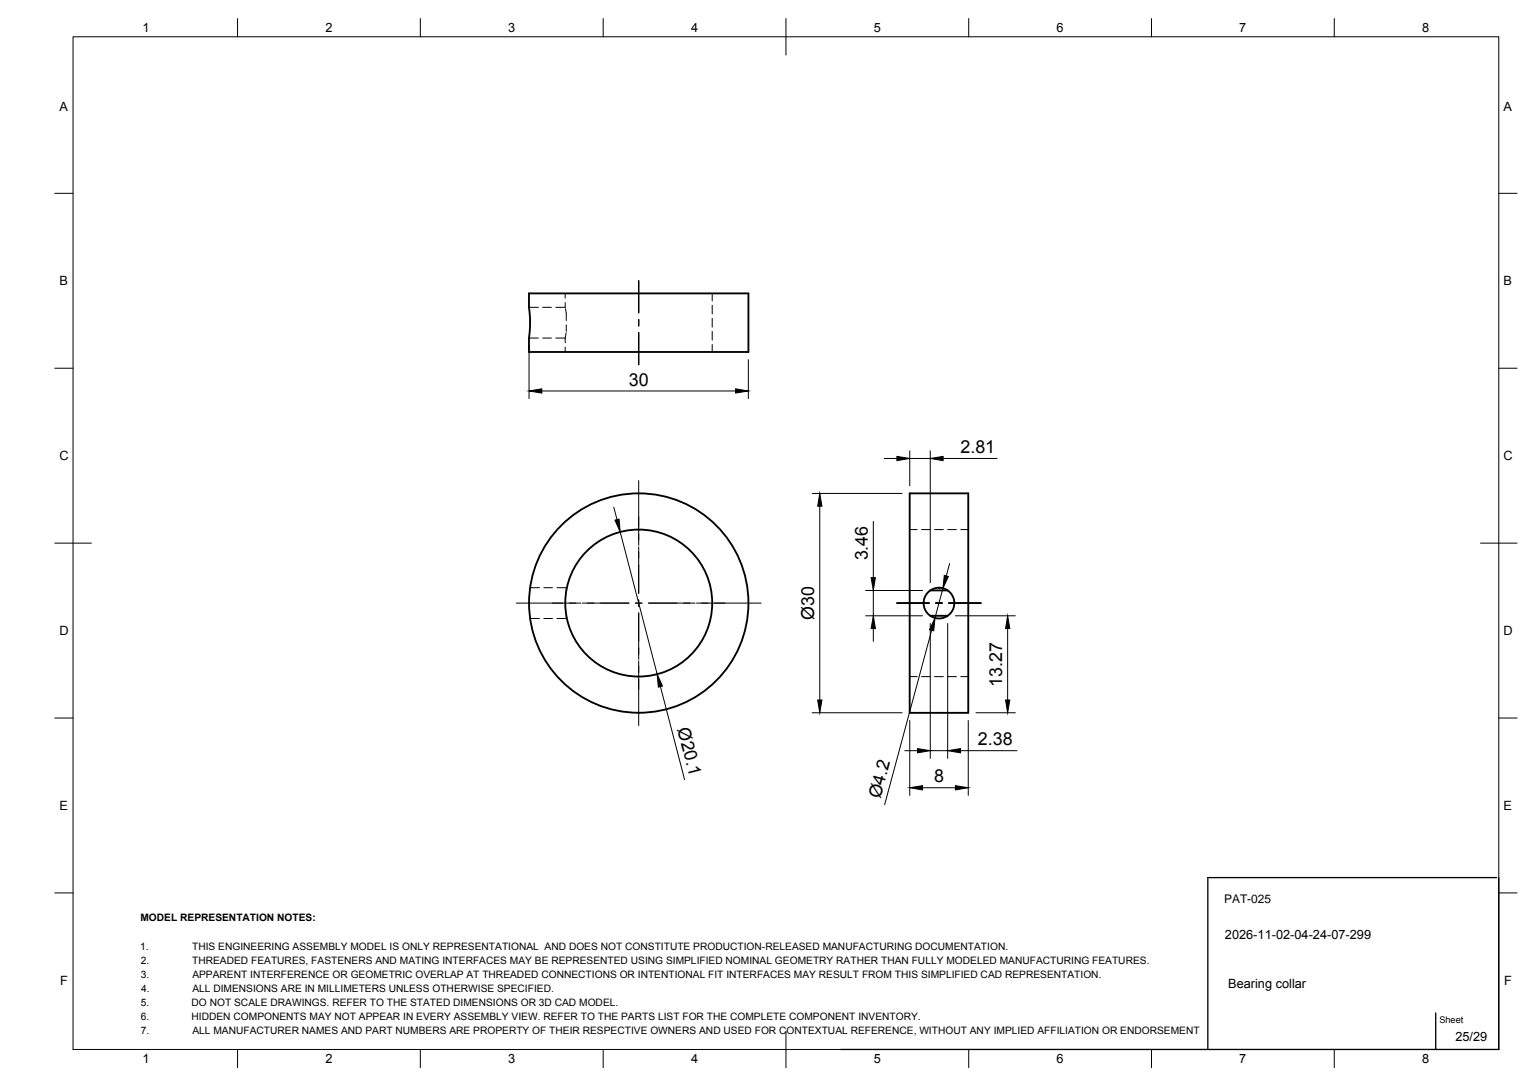
ISO-10303-21;
HEADER;
/* Generated by software containing ST-Developer
 * from STEP Tools, Inc. (www.steptools.com) 
 */

FILE_DESCRIPTION(
/* description */ ('Counter shaft with two pulleys and keyed hub'),
/* implementation_level */ '2;1');

FILE_NAME(
/* name */ 'Bearing collar.step',
/* time_stamp */ '2026-10-27T10:46:10-07:00',
/* author */ (''),
/* organization */ (''),
/* preprocessor_version */ 'ST-DEVELOPER v20.2',
/* originating_system */ 'Autodesk Translation Framework v15.17.0.0',
/* authorisation */ '');

FILE_SCHEMA (('AUTOMOTIVE_DESIGN { 1 0 10303 214 3 1 1 }'));
ENDSEC;

DATA;
#10=MECHANICAL_DESIGN_GEOMETRIC_PRESENTATION_REPRESENTATION('',(#309),#10821);
#212=B_SPLINE_CURVE_WITH_KNOTS('',3,(#9516,#9517,#9518,#9519,#9520,#9521,
#9522,#9523,#9524,#9525,#9526,#9527,#9528,#9529),.UNSPECIFIED.,.F.,.F.,
(4,2,2,2,2,2,4),(0.75600573798702,0.793568827564647,0.872922520054201,0.952276212543756,
1.03162990503331,1.11098359752287,1.14854668710049),.UNSPECIFIED.);
#213=B_SPLINE_CURVE_WITH_KNOTS('',3,(#9535,#9536,#9537,#9538,#9539,#9540,
#9541,#9542,#9543,#9544,#9545,#9546,#9547,#9548,#9549,#9550,#9551,#9552),
 .UNSPECIFIED.,.F.,.F.,(4,2,2,2,2,2,2,2,4),(0.,0.079216580773363,0.158433161546726,
0.23764869707457,0.316864232602414,0.396079768130259,0.475295303658103,
0.554511884431466,0.633728465204829),.UNSPECIFIED.);
#214=B_SPLINE_CURVE_WITH_KNOTS('',3,(#9553,#9554,#9555,#9556,#9557,#9558,
#9559,#9560,#9561,#9562,#9563,#9564,#9565,#9566,#9567,#9568,#9569,#9570),
 .UNSPECIFIED.,.F.,.F.,(4,2,2,2,2,2,2,2,4),(0.633728465204829,0.712945045978192,
0.792161626751555,0.871377162279399,0.950592697807244,1.02980823333509,
1.10902376886293,1.18824034963629,1.26745693040966),.UNSPECIFIED.);
#215=B_SPLINE_CURVE_WITH_KNOTS('',3,(#9573,#9574,#9575,#9576,#9577,#9578,
#9579,#9580,#9581,#9582,#9583,#9584,#9585,#9586),.UNSPECIFIED.,.F.,.F.,
(4,2,2,2,2,2,4),(0.121154929624515,0.158718019202143,0.238071711691697,
0.317425404181252,0.396779096670807,0.476132789160362,0.513695878737989),
 .UNSPECIFIED.);
#258=SHAPE_REPRESENTATION_RELATIONSHIP('SRR','None',#10946,#283);
#283=ADVANCED_BREP_SHAPE_REPRESENTATION('',(#334),#10814);
#309=STYLED_ITEM('',(#11135),#334);
#334=MANIFOLD_SOLID_BREP('Body1',#5593);
#409=FACE_BOUND('',#1130,.T.);
#410=FACE_BOUND('',#1132,.T.);
#411=FACE_BOUND('',#1134,.T.);
#412=FACE_BOUND('',#1136,.T.);
#532=PLANE('',#6178);
#533=PLANE('',#6183);
#534=PLANE('',#6190);
#535=PLANE('',#6191);
#743=FACE_OUTER_BOUND('',#1126,.T.);
#744=FACE_OUTER_BOUND('',#1127,.T.);
#745=FACE_OUTER_BOUND('',#1128,.T.);
#746=FACE_OUTER_BOUND('',#1129,.T.);
#747=FACE_OUTER_BOUND('',#1131,.T.);
#748=FACE_OUTER_BOUND('',#1133,.T.);
#749=FACE_OUTER_BOUND('',#1135,.T.);
#1126=EDGE_LOOP('',(#4269,#4270));
#1127=EDGE_LOOP('',(#4271,#4272,#4273,#4274,#4275,#4276,#4277,#4278,#4279));
#1128=EDGE_LOOP('',(#4280,#4281,#4282));
#1129=EDGE_LOOP('',(#4283,#4284,#4285,#4286));
#1130=EDGE_LOOP('',(#4287,#4288,#4289,#4290));
#1131=EDGE_LOOP('',(#4291,#4292,#4293,#4294));
#1132=EDGE_LOOP('',(#4295,#4296));
#1133=EDGE_LOOP('',(#4297));
#1134=EDGE_LOOP('',(#4298));
#1135=EDGE_LOOP('',(#4299));
#1136=EDGE_LOOP('',(#4300));
#1495=LINE('',#9512,#1884);
#1496=LINE('',#9533,#1885);
#1497=LINE('',#9588,#1886);
#1498=LINE('',#9593,#1887);
#1499=LINE('',#9599,#1888);
#1884=VECTOR('',#7351,1.);
#1885=VECTOR('',#7358,0.21);
#1886=VECTOR('',#7363,1.);
#1887=VECTOR('',#7368,1.005);
#1888=VECTOR('',#7375,1.5);
#2189=CIRCLE('',#6179,0.21);
#2190=CIRCLE('',#6181,0.21);
#2191=CIRCLE('',#6182,0.21);
#2192=CIRCLE('',#6185,1.005);
#2193=CIRCLE('',#6186,1.005);
#2194=CIRCLE('',#6188,1.5);
#2195=CIRCLE('',#6189,1.5);
#2604=VERTEX_POINT('',#9510);
#2605=VERTEX_POINT('',#9511);
#2606=VERTEX_POINT('',#9515);
#2607=VERTEX_POINT('',#9530);
#2608=VERTEX_POINT('',#9532);
#2609=VERTEX_POINT('',#9534);
#2610=VERTEX_POINT('',#9571);
#2611=VERTEX_POINT('',#9590);
#2612=VERTEX_POINT('',#9592);
#2613=VERTEX_POINT('',#9596);
#2614=VERTEX_POINT('',#9598);
#3207=EDGE_CURVE('',#2604,#2605,#1495,.T.);
#3208=EDGE_CURVE('',#2604,#2605,#2189,.T.);
#3209=EDGE_CURVE('',#2606,#2604,#212,.T.);
#3210=EDGE_CURVE('',#2607,#2606,#2190,.T.);
#3211=EDGE_CURVE('',#2607,#2608,#1496,.T.);
#3212=EDGE_CURVE('',#2609,#2608,#213,.T.);
#3213=EDGE_CURVE('',#2608,#2609,#214,.T.);
#3214=EDGE_CURVE('',#2610,#2607,#2191,.T.);
#3215=EDGE_CURVE('',#2605,#2610,#215,.T.);
#3216=EDGE_CURVE('',#2610,#2606,#1497,.T.);
#3217=EDGE_CURVE('',#2611,#2611,#2192,.T.);
#3218=EDGE_CURVE('',#2611,#2612,#1498,.T.);
#3219=EDGE_CURVE('',#2612,#2612,#2193,.T.);
#3220=EDGE_CURVE('',#2613,#2613,#2194,.T.);
#3221=EDGE_CURVE('',#2613,#2614,#1499,.T.);
#3222=EDGE_CURVE('',#2614,#2614,#2195,.T.);
#4269=ORIENTED_EDGE('',*,*,#3207,.F.);
#4270=ORIENTED_EDGE('',*,*,#3208,.T.);
#4271=ORIENTED_EDGE('',*,*,#3209,.F.);
#4272=ORIENTED_EDGE('',*,*,#3210,.F.);
#4273=ORIENTED_EDGE('',*,*,#3211,.T.);
#4274=ORIENTED_EDGE('',*,*,#3212,.F.);
#4275=ORIENTED_EDGE('',*,*,#3213,.F.);
#4276=ORIENTED_EDGE('',*,*,#3211,.F.);
#4277=ORIENTED_EDGE('',*,*,#3214,.F.);
#4278=ORIENTED_EDGE('',*,*,#3215,.F.);
#4279=ORIENTED_EDGE('',*,*,#3208,.F.);
#4280=ORIENTED_EDGE('',*,*,#3216,.F.);
#4281=ORIENTED_EDGE('',*,*,#3214,.T.);
#4282=ORIENTED_EDGE('',*,*,#3210,.T.);
#4283=ORIENTED_EDGE('',*,*,#3217,.F.);
#4284=ORIENTED_EDGE('',*,*,#3218,.T.);
#4285=ORIENTED_EDGE('',*,*,#3219,.T.);
#4286=ORIENTED_EDGE('',*,*,#3218,.F.);
#4287=ORIENTED_EDGE('',*,*,#3215,.T.);
#4288=ORIENTED_EDGE('',*,*,#3216,.T.);
#4289=ORIENTED_EDGE('',*,*,#3209,.T.);
#4290=ORIENTED_EDGE('',*,*,#3207,.T.);
#4291=ORIENTED_EDGE('',*,*,#3220,.F.);
#4292=ORIENTED_EDGE('',*,*,#3221,.T.);
#4293=ORIENTED_EDGE('',*,*,#3222,.T.);
#4294=ORIENTED_EDGE('',*,*,#3221,.F.);
#4295=ORIENTED_EDGE('',*,*,#3212,.T.);
#4296=ORIENTED_EDGE('',*,*,#3213,.T.);
#4297=ORIENTED_EDGE('',*,*,#3220,.T.);
#4298=ORIENTED_EDGE('',*,*,#3217,.T.);
#4299=ORIENTED_EDGE('',*,*,#3222,.F.);
#4300=ORIENTED_EDGE('',*,*,#3219,.F.);
#5162=CYLINDRICAL_SURFACE('',#6180,0.21);
#5163=CYLINDRICAL_SURFACE('',#6184,1.005);
#5164=CYLINDRICAL_SURFACE('',#6187,1.5);
#5414=ADVANCED_FACE('',(#743),#532,.T.);
#5415=ADVANCED_FACE('',(#744),#5162,.F.);
#5416=ADVANCED_FACE('',(#745),#533,.T.);
#5417=ADVANCED_FACE('',(#746,#409),#5163,.F.);
#5418=ADVANCED_FACE('',(#747,#410),#5164,.T.);
#5419=ADVANCED_FACE('',(#748,#411),#534,.T.);
#5420=ADVANCED_FACE('',(#749,#412),#535,.F.);
#5593=CLOSED_SHELL('',(#5414,#5415,#5416,#5417,#5418,#5419,#5420));
#6177=AXIS2_PLACEMENT_3D('',#9508,#7347,#7348);
#6178=AXIS2_PLACEMENT_3D('',#9509,#7349,#7350);
#6179=AXIS2_PLACEMENT_3D('',#9513,#7352,#7353);
#6180=AXIS2_PLACEMENT_3D('',#9514,#7354,#7355);
#6181=AXIS2_PLACEMENT_3D('',#9531,#7356,#7357);
#6182=AXIS2_PLACEMENT_3D('',#9572,#7359,#7360);
#6183=AXIS2_PLACEMENT_3D('',#9587,#7361,#7362);
#6184=AXIS2_PLACEMENT_3D('',#9589,#7364,#7365);
#6185=AXIS2_PLACEMENT_3D('',#9591,#7366,#7367);
#6186=AXIS2_PLACEMENT_3D('',#9594,#7369,#7370);
#6187=AXIS2_PLACEMENT_3D('',#9595,#7371,#7372);
#6188=AXIS2_PLACEMENT_3D('',#9597,#7373,#7374);
#6189=AXIS2_PLACEMENT_3D('',#9600,#7376,#7377);
#6190=AXIS2_PLACEMENT_3D('',#9601,#7378,#7379);
#6191=AXIS2_PLACEMENT_3D('',#9602,#7380,#7381);
#7347=DIRECTION('axis',(0.,0.,1.));
#7348=DIRECTION('refdir',(1.,0.,0.));
#7349=DIRECTION('center_axis',(0.,0.,1.));
#7350=DIRECTION('ref_axis',(1.,0.,0.));
#7351=DIRECTION('',(0.,1.,0.));
#7352=DIRECTION('center_axis',(0.,0.,1.));
#7353=DIRECTION('ref_axis',(1.,0.,0.));
#7354=DIRECTION('center_axis',(0.,0.,1.));
#7355=DIRECTION('ref_axis',(1.,0.,0.));
#7356=DIRECTION('center_axis',(0.,0.,1.));
#7357=DIRECTION('ref_axis',(1.,0.,0.));
#7358=DIRECTION('',(0.,0.,1.));
#7359=DIRECTION('center_axis',(0.,0.,1.));
#7360=DIRECTION('ref_axis',(1.,0.,0.));
#7361=DIRECTION('center_axis',(0.,0.,1.));
#7362=DIRECTION('ref_axis',(1.,0.,0.));
#7363=DIRECTION('',(0.,-1.,0.));
#7364=DIRECTION('center_axis',(0.,1.,0.));
#7365=DIRECTION('ref_axis',(1.,0.,0.));
#7366=DIRECTION('center_axis',(0.,-1.,0.));
#7367=DIRECTION('ref_axis',(1.,0.,0.));
#7368=DIRECTION('',(0.,-1.,0.));
#7369=DIRECTION('center_axis',(0.,-1.,0.));
#7370=DIRECTION('ref_axis',(1.,0.,0.));
#7371=DIRECTION('center_axis',(0.,1.,0.));
#7372=DIRECTION('ref_axis',(1.,0.,0.));
#7373=DIRECTION('center_axis',(0.,1.,0.));
#7374=DIRECTION('ref_axis',(1.,0.,0.));
#7375=DIRECTION('',(0.,-1.,0.));
#7376=DIRECTION('center_axis',(0.,1.,0.));
#7377=DIRECTION('ref_axis',(1.,0.,0.));
#7378=DIRECTION('center_axis',(0.,1.,0.));
#7379=DIRECTION('ref_axis',(1.,0.,0.));
#7380=DIRECTION('center_axis',(0.,1.,0.));
#7381=DIRECTION('ref_axis',(1.,0.,0.));
#9508=CARTESIAN_POINT('',(0.,0.,0.));
#9509=CARTESIAN_POINT('Origin',(0.,-1.25,5.52));
#9510=CARTESIAN_POINT('',(0.172988438920056,-1.36905880899792,5.52));
#9511=CARTESIAN_POINT('',(0.172988438920056,-1.13094119100209,5.52));
#9512=CARTESIAN_POINT('',(0.172988438920056,-1.65,5.52));
#9513=CARTESIAN_POINT('Origin',(0.,-1.25,5.52));
#9514=CARTESIAN_POINT('Origin',(0.,-1.25,5.52));
#9515=CARTESIAN_POINT('',(-0.172988438920056,-1.36905880899792,5.52));
#9516=CARTESIAN_POINT('Ctrl Pts',(-0.172988438920056,-1.36905880899792,
5.52));
#9517=CARTESIAN_POINT('Ctrl Pts',(-0.165594865311314,-1.37980142239529,
5.52129192197638));
#9518=CARTESIAN_POINT('Ctrl Pts',(-0.157297138725606,-1.38968770937274,
5.52265394943905));
#9519=CARTESIAN_POINT('Ctrl Pts',(-0.129892073845076,-1.41709277425327,
5.5267480843909));
#9520=CARTESIAN_POINT('Ctrl Pts',(-0.106330167759284,-1.43324205633295,
5.52969589327638));
#9521=CARTESIAN_POINT('Ctrl Pts',(-0.0546129046324105,-1.45469779396491,
5.53385029472357));
#9522=CARTESIAN_POINT('Ctrl Pts',(-0.0264512308298517,-1.46,5.535));
#9523=CARTESIAN_POINT('Ctrl Pts',(0.0264512308298516,-1.46,5.535));
#9524=CARTESIAN_POINT('Ctrl Pts',(0.0546129046324104,-1.45469779396491,
5.53385029472357));
#9525=CARTESIAN_POINT('Ctrl Pts',(0.106330167759284,-1.43324205633295,5.52969589327638));
#9526=CARTESIAN_POINT('Ctrl Pts',(0.129892073845076,-1.41709277425327,5.5267480843909));
#9527=CARTESIAN_POINT('Ctrl Pts',(0.157297138725606,-1.38968770937274,5.52265394943905));
#9528=CARTESIAN_POINT('Ctrl Pts',(0.165594865311314,-1.37980142239529,5.52129192197638));
#9529=CARTESIAN_POINT('Ctrl Pts',(0.172988438920056,-1.36905880899792,5.52));
#9530=CARTESIAN_POINT('',(-0.21,-1.25,5.52));
#9531=CARTESIAN_POINT('Origin',(0.,-1.25,5.52));
#9532=CARTESIAN_POINT('',(-0.21,-1.25,6.01522725533839));
#9533=CARTESIAN_POINT('',(-0.21,-1.25,5.52));
#9534=CARTESIAN_POINT('',(0.21,-1.25,6.01522725533839));
#9535=CARTESIAN_POINT('Ctrl Pts',(0.21,-1.25,6.01522725533839));
#9536=CARTESIAN_POINT('Ctrl Pts',(0.21,-1.27640552692445,6.01522725533839));
#9537=CARTESIAN_POINT('Ctrl Pts',(0.204715737269596,-1.30454707409071,6.01600415954412));
#9538=CARTESIAN_POINT('Ctrl Pts',(0.183273763036331,-1.35627626890513,6.01880073282317));
#9539=CARTESIAN_POINT('Ctrl Pts',(0.167117923970394,-1.37986692412796,6.02077897157582));
#9540=CARTESIAN_POINT('Ctrl Pts',(0.129867169887369,-1.41711767821098,6.02448481141327));
#9541=CARTESIAN_POINT('Ctrl Pts',(0.106276408305765,-1.43327371000135,6.02645455657129));
#9542=CARTESIAN_POINT('Ctrl Pts',(0.0545468514059002,-1.45471582482622,
6.02923165515645));
#9543=CARTESIAN_POINT('Ctrl Pts',(0.0264051785092814,-1.46,6.03));
#9544=CARTESIAN_POINT('Ctrl Pts',(-0.0264051785092814,-1.46,6.03));
#9545=CARTESIAN_POINT('Ctrl Pts',(-0.0545468514059001,-1.45471582482622,
6.02923165515645));
#9546=CARTESIAN_POINT('Ctrl Pts',(-0.106276408305765,-1.43327371000135,
6.02645455657129));
#9547=CARTESIAN_POINT('Ctrl Pts',(-0.129867169887369,-1.41711767821098,
6.02448481141327));
#9548=CARTESIAN_POINT('Ctrl Pts',(-0.167117923970394,-1.37986692412796,
6.02077897157582));
#9549=CARTESIAN_POINT('Ctrl Pts',(-0.183273763036331,-1.35627626890513,
6.01880073282317));
#9550=CARTESIAN_POINT('Ctrl Pts',(-0.204715737269596,-1.30454707409071,
6.01600415954412));
#9551=CARTESIAN_POINT('Ctrl Pts',(-0.21,-1.27640552692445,6.01522725533839));
#9552=CARTESIAN_POINT('Ctrl Pts',(-0.21,-1.25,6.01522725533839));
#9553=CARTESIAN_POINT('Ctrl Pts',(-0.21,-1.25,6.01522725533839));
#9554=CARTESIAN_POINT('Ctrl Pts',(-0.21,-1.22359447307555,6.01522725533839));
#9555=CARTESIAN_POINT('Ctrl Pts',(-0.204715737269596,-1.19545292590929,
6.01600415954412));
#9556=CARTESIAN_POINT('Ctrl Pts',(-0.183273763036331,-1.14372373109487,
6.01880073282317));
#9557=CARTESIAN_POINT('Ctrl Pts',(-0.167117923970394,-1.12013307587204,
6.02077897157582));
#9558=CARTESIAN_POINT('Ctrl Pts',(-0.129867169887369,-1.08288232178902,
6.02448481141327));
#9559=CARTESIAN_POINT('Ctrl Pts',(-0.106276408305765,-1.06672628999865,
6.02645455657129));
#9560=CARTESIAN_POINT('Ctrl Pts',(-0.0545468514059002,-1.04528417517378,
6.02923165515645));
#9561=CARTESIAN_POINT('Ctrl Pts',(-0.0264051785092814,-1.04,6.03));
#9562=CARTESIAN_POINT('Ctrl Pts',(0.0264051785092814,-1.04,6.03));
#9563=CARTESIAN_POINT('Ctrl Pts',(0.0545468514059001,-1.04528417517378,
6.02923165515645));
#9564=CARTESIAN_POINT('Ctrl Pts',(0.106276408305765,-1.06672628999865,6.02645455657129));
#9565=CARTESIAN_POINT('Ctrl Pts',(0.129867169887369,-1.08288232178902,6.02448481141327));
#9566=CARTESIAN_POINT('Ctrl Pts',(0.167117923970394,-1.12013307587204,6.02077897157582));
#9567=CARTESIAN_POINT('Ctrl Pts',(0.183273763036331,-1.14372373109487,6.01880073282317));
#9568=CARTESIAN_POINT('Ctrl Pts',(0.204715737269596,-1.19545292590929,6.01600415954412));
#9569=CARTESIAN_POINT('Ctrl Pts',(0.21,-1.22359447307555,6.01522725533839));
#9570=CARTESIAN_POINT('Ctrl Pts',(0.21,-1.25,6.01522725533839));
#9571=CARTESIAN_POINT('',(-0.172988438920056,-1.13094119100209,5.52));
#9572=CARTESIAN_POINT('Origin',(0.,-1.25,5.52));
#9573=CARTESIAN_POINT('Ctrl Pts',(0.172988438920056,-1.13094119100209,5.52));
#9574=CARTESIAN_POINT('Ctrl Pts',(0.165594865311315,-1.12019857760471,5.52129192197638));
#9575=CARTESIAN_POINT('Ctrl Pts',(0.157297138725606,-1.11031229062726,5.52265394943905));
#9576=CARTESIAN_POINT('Ctrl Pts',(0.129892073845076,-1.08290722574673,5.5267480843909));
#9577=CARTESIAN_POINT('Ctrl Pts',(0.106330167759284,-1.06675794366705,5.52969589327638));
#9578=CARTESIAN_POINT('Ctrl Pts',(0.0546129046324104,-1.04530220603509,
5.53385029472357));
#9579=CARTESIAN_POINT('Ctrl Pts',(0.0264512308298516,-1.04,5.535));
#9580=CARTESIAN_POINT('Ctrl Pts',(-0.0264512308298516,-1.04,5.535));
#9581=CARTESIAN_POINT('Ctrl Pts',(-0.0546129046324104,-1.04530220603509,
5.53385029472357));
#9582=CARTESIAN_POINT('Ctrl Pts',(-0.106330167759284,-1.06675794366705,
5.52969589327638));
#9583=CARTESIAN_POINT('Ctrl Pts',(-0.129892073845076,-1.08290722574673,
5.5267480843909));
#9584=CARTESIAN_POINT('Ctrl Pts',(-0.157297138725606,-1.11031229062726,
5.52265394943905));
#9585=CARTESIAN_POINT('Ctrl Pts',(-0.165594865311315,-1.12019857760471,
5.52129192197638));
#9586=CARTESIAN_POINT('Ctrl Pts',(-0.172988438920056,-1.13094119100209,
5.52));
#9587=CARTESIAN_POINT('Origin',(0.,-1.25,5.52));
#9588=CARTESIAN_POINT('',(-0.172988438920056,-1.65,5.52));
#9589=CARTESIAN_POINT('Origin',(0.,-1.65,4.53));
#9590=CARTESIAN_POINT('',(-1.005,-0.85,4.53));
#9591=CARTESIAN_POINT('Origin',(0.,-0.85,4.53));
#9592=CARTESIAN_POINT('',(-1.005,-1.65,4.53));
#9593=CARTESIAN_POINT('',(-1.005,-1.65,4.53));
#9594=CARTESIAN_POINT('Origin',(0.,-1.65,4.53));
#9595=CARTESIAN_POINT('Origin',(0.,-1.65,4.53));
#9596=CARTESIAN_POINT('',(-1.5,-0.85,4.53));
#9597=CARTESIAN_POINT('Origin',(0.,-0.85,4.53));
#9598=CARTESIAN_POINT('',(-1.5,-1.65,4.53));
#9599=CARTESIAN_POINT('',(-1.5,-1.65,4.53));
#9600=CARTESIAN_POINT('Origin',(0.,-1.65,4.53));
#9601=CARTESIAN_POINT('Origin',(0.,-0.85,4.53));
#9602=CARTESIAN_POINT('Origin',(0.,-1.65,4.53));
#10784=UNCERTAINTY_MEASURE_WITH_UNIT(LENGTH_MEASURE(0.001),#10822,
'DISTANCE_ACCURACY_VALUE',
'Maximum model space distance between geometric entities at asserted c
onnectivities');
#10791=UNCERTAINTY_MEASURE_WITH_UNIT(LENGTH_MEASURE(0.001),#10822,
'DISTANCE_ACCURACY_VALUE',
'Maximum model space distance between geometric entities at asserted c
onnectivities');
#10814=(
GEOMETRIC_REPRESENTATION_CONTEXT(3)
GLOBAL_UNCERTAINTY_ASSIGNED_CONTEXT((#10784))
GLOBAL_UNIT_ASSIGNED_CONTEXT((#10822,#10824,#10825))
REPRESENTATION_CONTEXT('','3D')
);
#10821=(
GEOMETRIC_REPRESENTATION_CONTEXT(3)
GLOBAL_UNCERTAINTY_ASSIGNED_CONTEXT((#10791))
GLOBAL_UNIT_ASSIGNED_CONTEXT((#10822,#10824,#10825))
REPRESENTATION_CONTEXT('','3D')
);
#10822=(
LENGTH_UNIT()
NAMED_UNIT(*)
SI_UNIT(.CENTI.,.METRE.)
);
#10824=(
NAMED_UNIT(*)
PLANE_ANGLE_UNIT()
SI_UNIT($,.RADIAN.)
);
#10825=(
NAMED_UNIT(*)
SI_UNIT($,.STERADIAN.)
SOLID_ANGLE_UNIT()
);
#10848=SHAPE_DEFINITION_REPRESENTATION(#10896,#10946);
#10896=PRODUCT_DEFINITION_SHAPE('',$,#10976);
#10946=SHAPE_REPRESENTATION('',(#6177),#10814);
#10953=PRODUCT_DEFINITION_CONTEXT('part definition',#11042,'design');
#10976=PRODUCT_DEFINITION('Bearing collar','Bearing collar',#11005,#10953);
#11005=PRODUCT_DEFINITION_FORMATION('',$,#11066);
#11042=APPLICATION_CONTEXT(
'Core Data for Automotive Mechanical Design Process');
#11043=PRODUCT_CONTEXT('part definition',#11042,'mechanical');
#11066=PRODUCT('Bearing collar','Bearing collar','Bearing collar',(#11043));
#11129=COLOUR_RGB('Grey',0.48,0.52,0.57);
#11130=FILL_AREA_STYLE_COLOUR('',#11129);
#11131=FILL_AREA_STYLE('',(#11130));
#11132=SURFACE_STYLE_FILL_AREA(#11131);
#11133=SURFACE_SIDE_STYLE('',(#11132));
#11134=SURFACE_STYLE_USAGE(.BOTH.,#11133);
#11135=PRESENTATION_STYLE_ASSIGNMENT((#11134));
ENDSEC;
END-ISO-10303-21;
